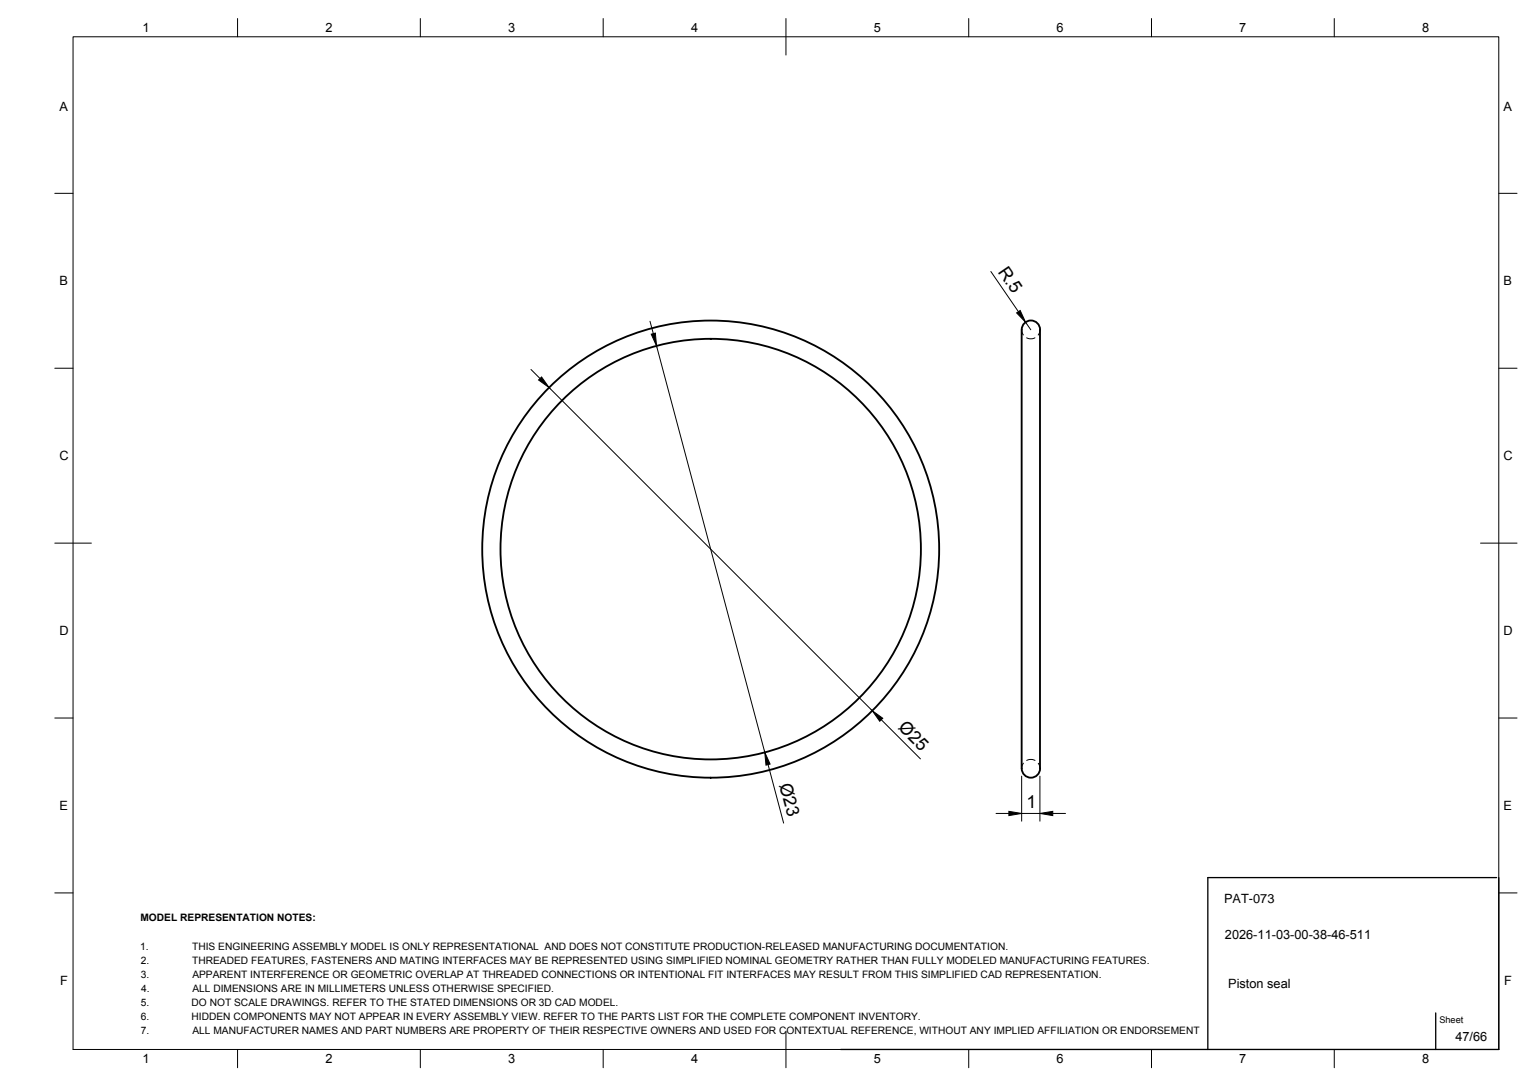
ISO-10303-21;
HEADER;
/* Generated by software containing ST-Developer
 * from STEP Tools, Inc. (www.steptools.com) 
 */

FILE_DESCRIPTION(
/* description */ ('Manual piston pump'),
/* implementation_level */ '2;1');

FILE_NAME(
/* name */ 'Piston seal.step',
/* time_stamp */ '2026-11-02T16:54:23-08:00',
/* author */ (''),
/* organization */ (''),
/* preprocessor_version */ 'ST-DEVELOPER v20.2',
/* originating_system */ 'Autodesk Translation Framework v15.17.0.0',
/* authorisation */ '');

FILE_SCHEMA (('AUTOMOTIVE_DESIGN { 1 0 10303 214 3 1 1 }'));
ENDSEC;

DATA;
#10=MECHANICAL_DESIGN_GEOMETRIC_PRESENTATION_REPRESENTATION('',(#738),#19043);
#561=TOROIDAL_SURFACE('',#11098,1.2,0.05);
#604=SHAPE_REPRESENTATION_RELATIONSHIP('SRR','None',#19353,#667);
#667=ADVANCED_BREP_SHAPE_REPRESENTATION('',(#807),#19020);
#738=STYLED_ITEM('',(#19661),#807);
#807=MANIFOLD_SOLID_BREP('Body1',#9525);
#1714=FACE_OUTER_BOUND('',#2467,.T.);
#2467=EDGE_LOOP('',(#7973,#7974,#7975,#7976));
#3036=CIRCLE('',#11099,0.05);
#3037=CIRCLE('',#11100,1.15);
#4927=VERTEX_POINT('',#17993);
#5973=EDGE_CURVE('',#4927,#4927,#3036,.T.);
#5974=EDGE_CURVE('',#4927,#4927,#3037,.T.);
#7973=ORIENTED_EDGE('',*,*,#5973,.F.);
#7974=ORIENTED_EDGE('',*,*,#5974,.T.);
#7975=ORIENTED_EDGE('',*,*,#5973,.T.);
#7976=ORIENTED_EDGE('',*,*,#5974,.F.);
#9319=ADVANCED_FACE('',(#1714),#561,.T.);
#9525=CLOSED_SHELL('',(#9319));
#11097=AXIS2_PLACEMENT_3D('',#17991,#13634,#13635);
#11098=AXIS2_PLACEMENT_3D('',#17992,#13636,#13637);
#11099=AXIS2_PLACEMENT_3D('',#17994,#13638,#13639);
#11100=AXIS2_PLACEMENT_3D('',#17995,#13640,#13641);
#13634=DIRECTION('axis',(0.,0.,1.));
#13635=DIRECTION('refdir',(1.,0.,0.));
#13636=DIRECTION('center_axis',(0.,-1.,0.));
#13637=DIRECTION('ref_axis',(0.,0.,-1.));
#13638=DIRECTION('center_axis',(-1.,0.,-1.22464679914735E-16));
#13639=DIRECTION('ref_axis',(-1.22464679914735E-16,0.,1.));
#13640=DIRECTION('center_axis',(0.,1.,0.));
#13641=DIRECTION('ref_axis',(0.,0.,-1.));
#17991=CARTESIAN_POINT('',(0.,0.,0.));
#17992=CARTESIAN_POINT('Origin',(0.,2.95,4.5));
#17993=CARTESIAN_POINT('',(-1.40834381901946E-16,2.95,5.65));
#17994=CARTESIAN_POINT('Origin',(-1.46957615897682E-16,2.95,5.7));
#17995=CARTESIAN_POINT('Origin',(0.,2.95,4.5));
#18949=UNCERTAINTY_MEASURE_WITH_UNIT(LENGTH_MEASURE(0.001),#19044,
'DISTANCE_ACCURACY_VALUE',
'Maximum model space distance between geometric entities at asserted c
onnectivities');
#18972=UNCERTAINTY_MEASURE_WITH_UNIT(LENGTH_MEASURE(0.001),#19044,
'DISTANCE_ACCURACY_VALUE',
'Maximum model space distance between geometric entities at asserted c
onnectivities');
#19020=(
GEOMETRIC_REPRESENTATION_CONTEXT(3)
GLOBAL_UNCERTAINTY_ASSIGNED_CONTEXT((#18949))
GLOBAL_UNIT_ASSIGNED_CONTEXT((#19044,#19046,#19047))
REPRESENTATION_CONTEXT('','3D')
);
#19043=(
GEOMETRIC_REPRESENTATION_CONTEXT(3)
GLOBAL_UNCERTAINTY_ASSIGNED_CONTEXT((#18972))
GLOBAL_UNIT_ASSIGNED_CONTEXT((#19044,#19046,#19047))
REPRESENTATION_CONTEXT('','3D')
);
#19044=(
LENGTH_UNIT()
NAMED_UNIT(*)
SI_UNIT(.CENTI.,.METRE.)
);
#19046=(
NAMED_UNIT(*)
PLANE_ANGLE_UNIT()
SI_UNIT($,.RADIAN.)
);
#19047=(
NAMED_UNIT(*)
SI_UNIT($,.STERADIAN.)
SOLID_ANGLE_UNIT()
);
#19095=SHAPE_DEFINITION_REPRESENTATION(#19172,#19353);
#19172=PRODUCT_DEFINITION_SHAPE('',$,#19424);
#19353=SHAPE_REPRESENTATION('',(#11097),#19020);
#19376=PRODUCT_DEFINITION_CONTEXT('part definition',#19588,'design');
#19424=PRODUCT_DEFINITION('2026-11-03-00-38-46-511','Piston seal',#19494,
#19376);
#19494=PRODUCT_DEFINITION_FORMATION('',$,#19637);
#19588=APPLICATION_CONTEXT(
'Core Data for Automotive Mechanical Design Process');
#19589=PRODUCT_CONTEXT('part definition',#19588,'mechanical');
#19637=PRODUCT('2026-11-03-00-38-46-511','Piston seal','Piston seal',(#19589));
#19661=PRESENTATION_STYLE_ASSIGNMENT((#19667));
#19667=SURFACE_STYLE_USAGE(.BOTH.,#19673);
#19673=SURFACE_SIDE_STYLE('',(#19679));
#19679=SURFACE_STYLE_FILL_AREA(#19685);
#19685=FILL_AREA_STYLE('CAD Library Painted - Engineering blue',(#19691));
#19691=FILL_AREA_STYLE_COLOUR('CAD Library Painted - Engineering blue',
#19697);
#19697=COLOUR_RGB('CAD Library Painted - Engineering blue',0.12156862745098,
0.356862745098039,0.6);
ENDSEC;
END-ISO-10303-21;
